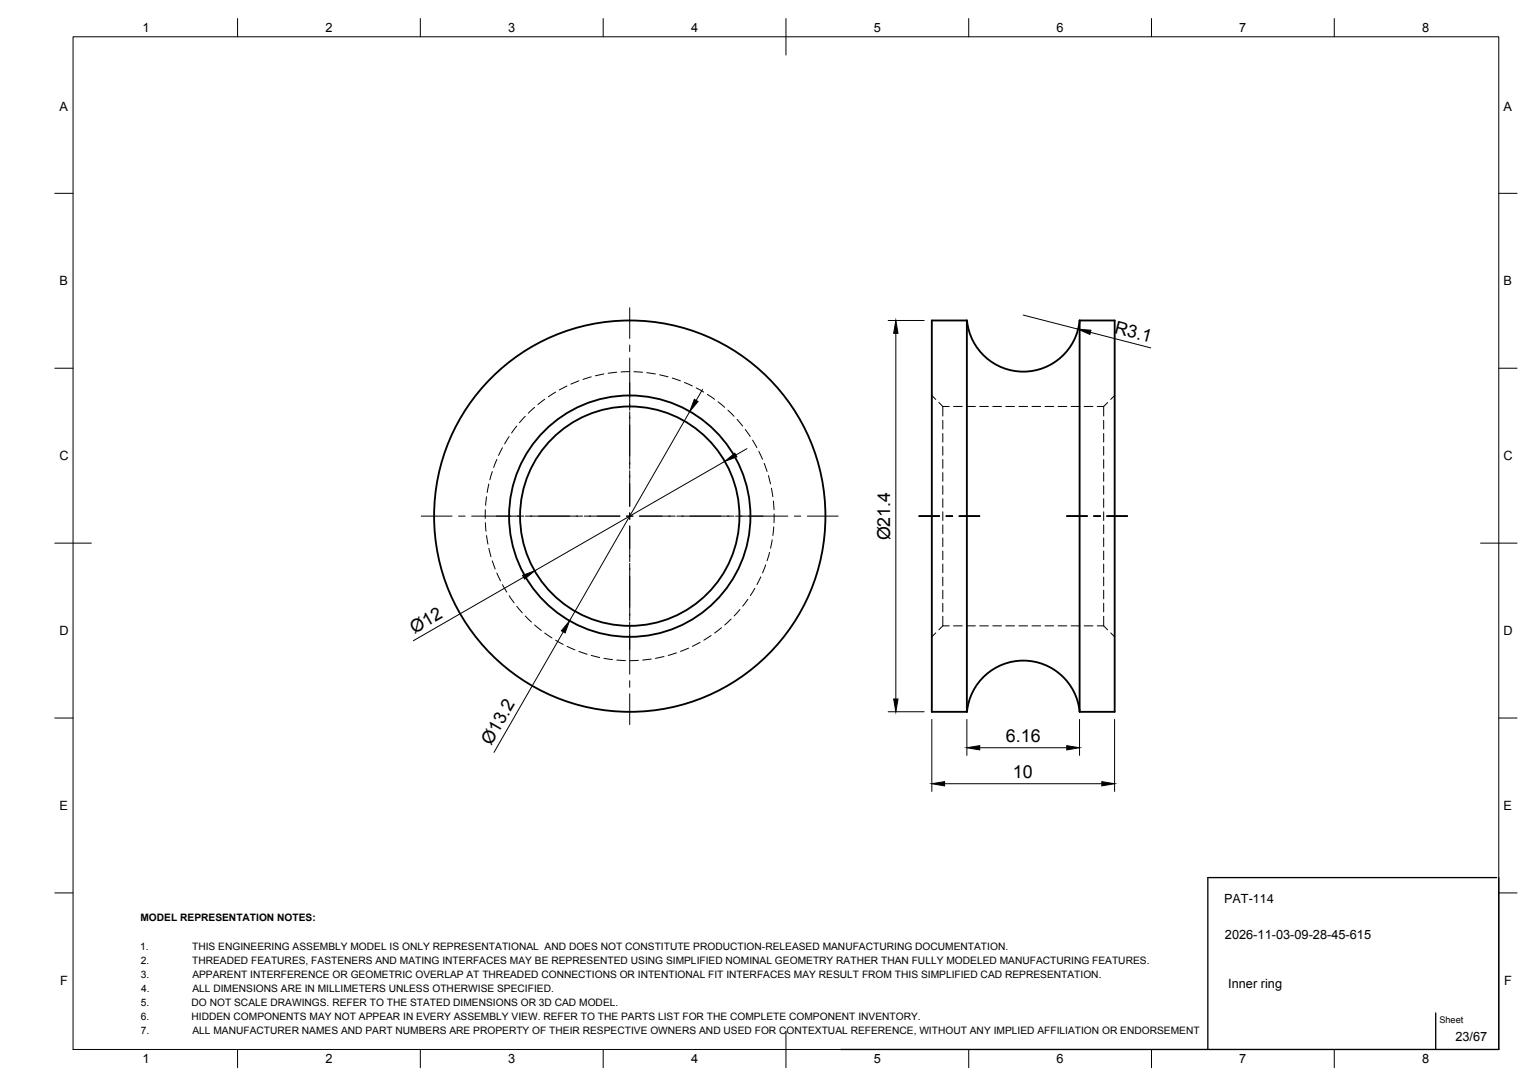
ISO-10303-21;
HEADER;
/* Generated by software containing ST-Developer
 * from STEP Tools, Inc. (www.steptools.com) 
 */

FILE_DESCRIPTION(
/* description */ ('Two-stage gear reducer in split housing'),
/* implementation_level */ '2;1');

FILE_NAME(
/* name */ 'Inner ring.step',
/* time_stamp */ '2026-10-28T03:22:31-07:00',
/* author */ (''),
/* organization */ (''),
/* preprocessor_version */ 'ST-DEVELOPER v20.2',
/* originating_system */ 'Autodesk Translation Framework v15.17.0.0',
/* authorisation */ '');

FILE_SCHEMA (('AUTOMOTIVE_DESIGN { 1 0 10303 214 3 1 1 }'));
ENDSEC;

DATA;
#10=MECHANICAL_DESIGN_GEOMETRIC_PRESENTATION_REPRESENTATION('',(#1251),#73366);
#1097=TOROIDAL_SURFACE('',#17418,1.1,0.309556);
#1104=CONICAL_SURFACE('',#17429,0.63,0.785398163397448);
#1105=CONICAL_SURFACE('',#17436,0.63,0.785398163397448);
#1139=SHAPE_REPRESENTATION_RELATIONSHIP('SRR','None',#73627,#1195);
#1195=ADVANCED_BREP_SHAPE_REPRESENTATION('',(#1321),#73323);
#1251=STYLED_ITEM('',(#73988),#1321);
#1321=MANIFOLD_SOLID_BREP('Body1',#16140);
#1519=FACE_BOUND('',#3363,.T.);
#1520=FACE_BOUND('',#3366,.T.);
#1755=PLANE('',#17431);
#1756=PLANE('',#17434);
#2300=FACE_OUTER_BOUND('',#3358,.T.);
#2301=FACE_OUTER_BOUND('',#3359,.T.);
#2302=FACE_OUTER_BOUND('',#3360,.T.);
#2303=FACE_OUTER_BOUND('',#3361,.T.);
#2304=FACE_OUTER_BOUND('',#3362,.T.);
#2305=FACE_OUTER_BOUND('',#3364,.T.);
#2306=FACE_OUTER_BOUND('',#3365,.T.);
#2307=FACE_OUTER_BOUND('',#3367,.T.);
#3358=EDGE_LOOP('',(#11815,#11816,#11817,#11818,#11819,#11820));
#3359=EDGE_LOOP('',(#11821,#11822,#11823,#11824,#11825));
#3360=EDGE_LOOP('',(#11826,#11827,#11828,#11829));
#3361=EDGE_LOOP('',(#11830,#11831,#11832,#11833));
#3362=EDGE_LOOP('',(#11834));
#3363=EDGE_LOOP('',(#11835));
#3364=EDGE_LOOP('',(#11836,#11837,#11838,#11839,#11840));
#3365=EDGE_LOOP('',(#11841));
#3366=EDGE_LOOP('',(#11842));
#3367=EDGE_LOOP('',(#11843,#11844,#11845,#11846));
#4423=LINE('',#24194,#5447);
#4424=LINE('',#24200,#5448);
#4425=LINE('',#24204,#5449);
#4426=LINE('',#24210,#5450);
#4427=LINE('',#24215,#5451);
#5447=VECTOR('',#20051,1.070235);
#5448=VECTOR('',#20058,0.6);
#5449=VECTOR('',#20063,0.63);
#5450=VECTOR('',#20072,1.070235);
#5451=VECTOR('',#20079,0.63);
#6391=CIRCLE('',#17419,1.070235);
#6392=CIRCLE('',#17420,1.070235);
#6393=CIRCLE('',#17421,0.309556);
#6394=CIRCLE('',#17422,1.070235);
#6395=CIRCLE('',#17423,1.070235);
#6396=CIRCLE('',#17425,1.070235);
#6397=CIRCLE('',#17427,0.6);
#6398=CIRCLE('',#17428,0.6);
#6399=CIRCLE('',#17430,0.66);
#6400=CIRCLE('',#17433,1.070235);
#6401=CIRCLE('',#17435,0.66);
#7259=VERTEX_POINT('',#24183);
#7260=VERTEX_POINT('',#24184);
#7261=VERTEX_POINT('',#24187);
#7262=VERTEX_POINT('',#24189);
#7263=VERTEX_POINT('',#24193);
#7264=VERTEX_POINT('',#24197);
#7265=VERTEX_POINT('',#24199);
#7266=VERTEX_POINT('',#24203);
#7267=VERTEX_POINT('',#24208);
#7268=VERTEX_POINT('',#24212);
#8961=EDGE_CURVE('',#7259,#7260,#6391,.T.);
#8962=EDGE_CURVE('',#7260,#7259,#6392,.T.);
#8963=EDGE_CURVE('',#7260,#7261,#6393,.T.);
#8964=EDGE_CURVE('',#7262,#7261,#6394,.T.);
#8965=EDGE_CURVE('',#7261,#7262,#6395,.T.);
#8966=EDGE_CURVE('',#7262,#7263,#4423,.T.);
#8967=EDGE_CURVE('',#7263,#7263,#6396,.T.);
#8968=EDGE_CURVE('',#7264,#7264,#6397,.T.);
#8969=EDGE_CURVE('',#7264,#7265,#4424,.T.);
#8970=EDGE_CURVE('',#7265,#7265,#6398,.T.);
#8971=EDGE_CURVE('',#7265,#7266,#4425,.T.);
#8972=EDGE_CURVE('',#7266,#7266,#6399,.T.);
#8973=EDGE_CURVE('',#7267,#7267,#6400,.T.);
#8974=EDGE_CURVE('',#7267,#7259,#4426,.T.);
#8975=EDGE_CURVE('',#7268,#7268,#6401,.T.);
#8976=EDGE_CURVE('',#7268,#7264,#4427,.T.);
#11815=ORIENTED_EDGE('',*,*,#8961,.F.);
#11816=ORIENTED_EDGE('',*,*,#8962,.F.);
#11817=ORIENTED_EDGE('',*,*,#8963,.T.);
#11818=ORIENTED_EDGE('',*,*,#8964,.F.);
#11819=ORIENTED_EDGE('',*,*,#8965,.F.);
#11820=ORIENTED_EDGE('',*,*,#8963,.F.);
#11821=ORIENTED_EDGE('',*,*,#8964,.T.);
#11822=ORIENTED_EDGE('',*,*,#8965,.T.);
#11823=ORIENTED_EDGE('',*,*,#8966,.T.);
#11824=ORIENTED_EDGE('',*,*,#8967,.T.);
#11825=ORIENTED_EDGE('',*,*,#8966,.F.);
#11826=ORIENTED_EDGE('',*,*,#8968,.T.);
#11827=ORIENTED_EDGE('',*,*,#8969,.T.);
#11828=ORIENTED_EDGE('',*,*,#8970,.F.);
#11829=ORIENTED_EDGE('',*,*,#8969,.F.);
#11830=ORIENTED_EDGE('',*,*,#8970,.T.);
#11831=ORIENTED_EDGE('',*,*,#8971,.T.);
#11832=ORIENTED_EDGE('',*,*,#8972,.F.);
#11833=ORIENTED_EDGE('',*,*,#8971,.F.);
#11834=ORIENTED_EDGE('',*,*,#8967,.F.);
#11835=ORIENTED_EDGE('',*,*,#8972,.T.);
#11836=ORIENTED_EDGE('',*,*,#8973,.F.);
#11837=ORIENTED_EDGE('',*,*,#8974,.T.);
#11838=ORIENTED_EDGE('',*,*,#8961,.T.);
#11839=ORIENTED_EDGE('',*,*,#8962,.T.);
#11840=ORIENTED_EDGE('',*,*,#8974,.F.);
#11841=ORIENTED_EDGE('',*,*,#8973,.T.);
#11842=ORIENTED_EDGE('',*,*,#8975,.F.);
#11843=ORIENTED_EDGE('',*,*,#8975,.T.);
#11844=ORIENTED_EDGE('',*,*,#8976,.T.);
#11845=ORIENTED_EDGE('',*,*,#8968,.F.);
#11846=ORIENTED_EDGE('',*,*,#8976,.F.);
#15049=CYLINDRICAL_SURFACE('',#17424,1.070235);
#15050=CYLINDRICAL_SURFACE('',#17426,0.6);
#15051=CYLINDRICAL_SURFACE('',#17432,1.070235);
#15507=ADVANCED_FACE('',(#2300),#1097,.F.);
#15508=ADVANCED_FACE('',(#2301),#15049,.T.);
#15509=ADVANCED_FACE('',(#2302),#15050,.F.);
#15510=ADVANCED_FACE('',(#2303),#1104,.F.);
#15511=ADVANCED_FACE('',(#2304,#1519),#1755,.T.);
#15512=ADVANCED_FACE('',(#2305),#15051,.T.);
#15513=ADVANCED_FACE('',(#2306,#1520),#1756,.T.);
#15514=ADVANCED_FACE('',(#2307),#1105,.F.);
#16140=CLOSED_SHELL('',(#15507,#15508,#15509,#15510,#15511,#15512,#15513,
#15514));
#17417=AXIS2_PLACEMENT_3D('',#24181,#20035,#20036);
#17418=AXIS2_PLACEMENT_3D('',#24182,#20037,#20038);
#17419=AXIS2_PLACEMENT_3D('',#24185,#20039,#20040);
#17420=AXIS2_PLACEMENT_3D('',#24186,#20041,#20042);
#17421=AXIS2_PLACEMENT_3D('',#24188,#20043,#20044);
#17422=AXIS2_PLACEMENT_3D('',#24190,#20045,#20046);
#17423=AXIS2_PLACEMENT_3D('',#24191,#20047,#20048);
#17424=AXIS2_PLACEMENT_3D('',#24192,#20049,#20050);
#17425=AXIS2_PLACEMENT_3D('',#24195,#20052,#20053);
#17426=AXIS2_PLACEMENT_3D('',#24196,#20054,#20055);
#17427=AXIS2_PLACEMENT_3D('',#24198,#20056,#20057);
#17428=AXIS2_PLACEMENT_3D('',#24201,#20059,#20060);
#17429=AXIS2_PLACEMENT_3D('',#24202,#20061,#20062);
#17430=AXIS2_PLACEMENT_3D('',#24205,#20064,#20065);
#17431=AXIS2_PLACEMENT_3D('',#24206,#20066,#20067);
#17432=AXIS2_PLACEMENT_3D('',#24207,#20068,#20069);
#17433=AXIS2_PLACEMENT_3D('',#24209,#20070,#20071);
#17434=AXIS2_PLACEMENT_3D('',#24211,#20073,#20074);
#17435=AXIS2_PLACEMENT_3D('',#24213,#20075,#20076);
#17436=AXIS2_PLACEMENT_3D('',#24214,#20077,#20078);
#20035=DIRECTION('axis',(0.,0.,1.));
#20036=DIRECTION('refdir',(1.,0.,0.));
#20037=DIRECTION('center_axis',(0.,-1.,0.));
#20038=DIRECTION('ref_axis',(0.,0.,-1.));
#20039=DIRECTION('center_axis',(0.,-1.,0.));
#20040=DIRECTION('ref_axis',(1.,0.,0.));
#20041=DIRECTION('center_axis',(0.,-1.,0.));
#20042=DIRECTION('ref_axis',(1.,0.,0.));
#20043=DIRECTION('center_axis',(1.,0.,1.22464679914735E-16));
#20044=DIRECTION('ref_axis',(-1.22464679914735E-16,0.,1.));
#20045=DIRECTION('center_axis',(0.,1.,0.));
#20046=DIRECTION('ref_axis',(1.,0.,0.));
#20047=DIRECTION('center_axis',(0.,1.,0.));
#20048=DIRECTION('ref_axis',(1.,0.,0.));
#20049=DIRECTION('center_axis',(0.,-1.,0.));
#20050=DIRECTION('ref_axis',(1.,0.,0.));
#20051=DIRECTION('',(0.,1.,0.));
#20052=DIRECTION('center_axis',(0.,-1.,0.));
#20053=DIRECTION('ref_axis',(1.,0.,0.));
#20054=DIRECTION('center_axis',(0.,-1.,0.));
#20055=DIRECTION('ref_axis',(1.,0.,0.));
#20056=DIRECTION('center_axis',(0.,-1.,0.));
#20057=DIRECTION('ref_axis',(1.,0.,0.));
#20058=DIRECTION('',(0.,1.,0.));
#20059=DIRECTION('center_axis',(0.,-1.,0.));
#20060=DIRECTION('ref_axis',(1.,0.,0.));
#20061=DIRECTION('center_axis',(0.,1.,0.));
#20062=DIRECTION('ref_axis',(1.,0.,0.));
#20063=DIRECTION('',(-0.707106781186548,0.707106781186547,-8.65956056235493E-17));
#20064=DIRECTION('center_axis',(0.,-1.,0.));
#20065=DIRECTION('ref_axis',(1.,0.,0.));
#20066=DIRECTION('center_axis',(0.,1.,0.));
#20067=DIRECTION('ref_axis',(0.,0.,1.));
#20068=DIRECTION('center_axis',(0.,-1.,0.));
#20069=DIRECTION('ref_axis',(1.,0.,0.));
#20070=DIRECTION('center_axis',(0.,-1.,0.));
#20071=DIRECTION('ref_axis',(1.,0.,0.));
#20072=DIRECTION('',(0.,1.,0.));
#20073=DIRECTION('center_axis',(0.,-1.,0.));
#20074=DIRECTION('ref_axis',(0.,0.,-1.));
#20075=DIRECTION('center_axis',(0.,-1.,0.));
#20076=DIRECTION('ref_axis',(1.,0.,0.));
#20077=DIRECTION('center_axis',(0.,-1.,0.));
#20078=DIRECTION('ref_axis',(1.,0.,0.));
#20079=DIRECTION('',(0.707106781186548,0.707106781186547,8.65956056235493E-17));
#24181=CARTESIAN_POINT('',(0.,0.,0.));
#24182=CARTESIAN_POINT('Origin',(0.,0.,0.));
#24183=CARTESIAN_POINT('',(-1.070235,-0.308121667383195,-1.31065986708547E-16));
#24184=CARTESIAN_POINT('',(-1.31065986708547E-16,-0.308121667383195,1.070235));
#24185=CARTESIAN_POINT('Origin',(0.,-0.308121667383195,0.));
#24186=CARTESIAN_POINT('Origin',(0.,-0.308121667383195,0.));
#24187=CARTESIAN_POINT('',(-1.31065986708547E-16,0.308121667383195,1.070235));
#24188=CARTESIAN_POINT('Origin',(-1.34711147906209E-16,0.,1.1));
#24189=CARTESIAN_POINT('',(-1.070235,0.308121667383195,1.31065986708547E-16));
#24190=CARTESIAN_POINT('Origin',(0.,0.308121667383195,0.));
#24191=CARTESIAN_POINT('Origin',(0.,0.308121667383195,0.));
#24192=CARTESIAN_POINT('Origin',(0.,0.,0.));
#24193=CARTESIAN_POINT('',(-1.070235,0.5,-1.31065986708547E-16));
#24194=CARTESIAN_POINT('',(-1.070235,0.,-1.31065986708547E-16));
#24195=CARTESIAN_POINT('Origin',(0.,0.5,0.));
#24196=CARTESIAN_POINT('Origin',(0.,0.,0.));
#24197=CARTESIAN_POINT('',(-0.6,-0.44,-7.34788079488412E-17));
#24198=CARTESIAN_POINT('Origin',(0.,-0.44,0.));
#24199=CARTESIAN_POINT('',(-0.6,0.44,-7.34788079488412E-17));
#24200=CARTESIAN_POINT('',(-0.6,0.,-7.34788079488412E-17));
#24201=CARTESIAN_POINT('Origin',(0.,0.44,0.));
#24202=CARTESIAN_POINT('Origin',(0.,0.47,0.));
#24203=CARTESIAN_POINT('',(-0.66,0.5,-8.08266887437253E-17));
#24204=CARTESIAN_POINT('',(-0.63,0.47,-7.71527483462832E-17));
#24205=CARTESIAN_POINT('Origin',(0.,0.5,0.));
#24206=CARTESIAN_POINT('Origin',(1.070235,0.5,0.));
#24207=CARTESIAN_POINT('Origin',(0.,0.,0.));
#24208=CARTESIAN_POINT('',(-1.070235,-0.5,-1.31065986708547E-16));
#24209=CARTESIAN_POINT('Origin',(0.,-0.5,0.));
#24210=CARTESIAN_POINT('',(-1.070235,0.,-1.31065986708547E-16));
#24211=CARTESIAN_POINT('Origin',(0.66,-0.5,0.));
#24212=CARTESIAN_POINT('',(-0.66,-0.5,-8.08266887437253E-17));
#24213=CARTESIAN_POINT('Origin',(0.,-0.5,0.));
#24214=CARTESIAN_POINT('Origin',(0.,-0.47,0.));
#24215=CARTESIAN_POINT('',(-0.63,-0.47,-7.71527483462832E-17));
#73259=UNCERTAINTY_MEASURE_WITH_UNIT(LENGTH_MEASURE(0.001),#73367,
'DISTANCE_ACCURACY_VALUE',
'Maximum model space distance between geometric entities at asserted c
onnectivities');
#73302=UNCERTAINTY_MEASURE_WITH_UNIT(LENGTH_MEASURE(0.001),#73367,
'DISTANCE_ACCURACY_VALUE',
'Maximum model space distance between geometric entities at asserted c
onnectivities');
#73323=(
GEOMETRIC_REPRESENTATION_CONTEXT(3)
GLOBAL_UNCERTAINTY_ASSIGNED_CONTEXT((#73259))
GLOBAL_UNIT_ASSIGNED_CONTEXT((#73367,#73369,#73370))
REPRESENTATION_CONTEXT('','3D')
);
#73366=(
GEOMETRIC_REPRESENTATION_CONTEXT(3)
GLOBAL_UNCERTAINTY_ASSIGNED_CONTEXT((#73302))
GLOBAL_UNIT_ASSIGNED_CONTEXT((#73367,#73369,#73370))
REPRESENTATION_CONTEXT('','3D')
);
#73367=(
LENGTH_UNIT()
NAMED_UNIT(*)
SI_UNIT(.CENTI.,.METRE.)
);
#73369=(
NAMED_UNIT(*)
PLANE_ANGLE_UNIT()
SI_UNIT($,.RADIAN.)
);
#73370=(
NAMED_UNIT(*)
SI_UNIT($,.STERADIAN.)
SOLID_ANGLE_UNIT()
);
#73391=SHAPE_DEFINITION_REPRESENTATION(#73454,#73627);
#73454=PRODUCT_DEFINITION_SHAPE('',$,#73691);
#73627=SHAPE_REPRESENTATION('',(#17417),#73323);
#73670=PRODUCT_DEFINITION_CONTEXT('part definition',#73861,'design');
#73691=PRODUCT_DEFINITION('Inner ring','Inner ring',#73754,#73670);
#73754=PRODUCT_DEFINITION_FORMATION('',$,#73883);
#73861=APPLICATION_CONTEXT(
'Core Data for Automotive Mechanical Design Process');
#73862=PRODUCT_CONTEXT('part definition',#73861,'mechanical');
#73883=PRODUCT('Inner ring','Inner ring','Inner ring',(#73862));
#73982=COLOUR_RGB('Grey',0.48,0.52,0.57);
#73983=FILL_AREA_STYLE_COLOUR('',#73982);
#73984=FILL_AREA_STYLE('',(#73983));
#73985=SURFACE_STYLE_FILL_AREA(#73984);
#73986=SURFACE_SIDE_STYLE('',(#73985));
#73987=SURFACE_STYLE_USAGE(.BOTH.,#73986);
#73988=PRESENTATION_STYLE_ASSIGNMENT((#73987));
ENDSEC;
END-ISO-10303-21;
